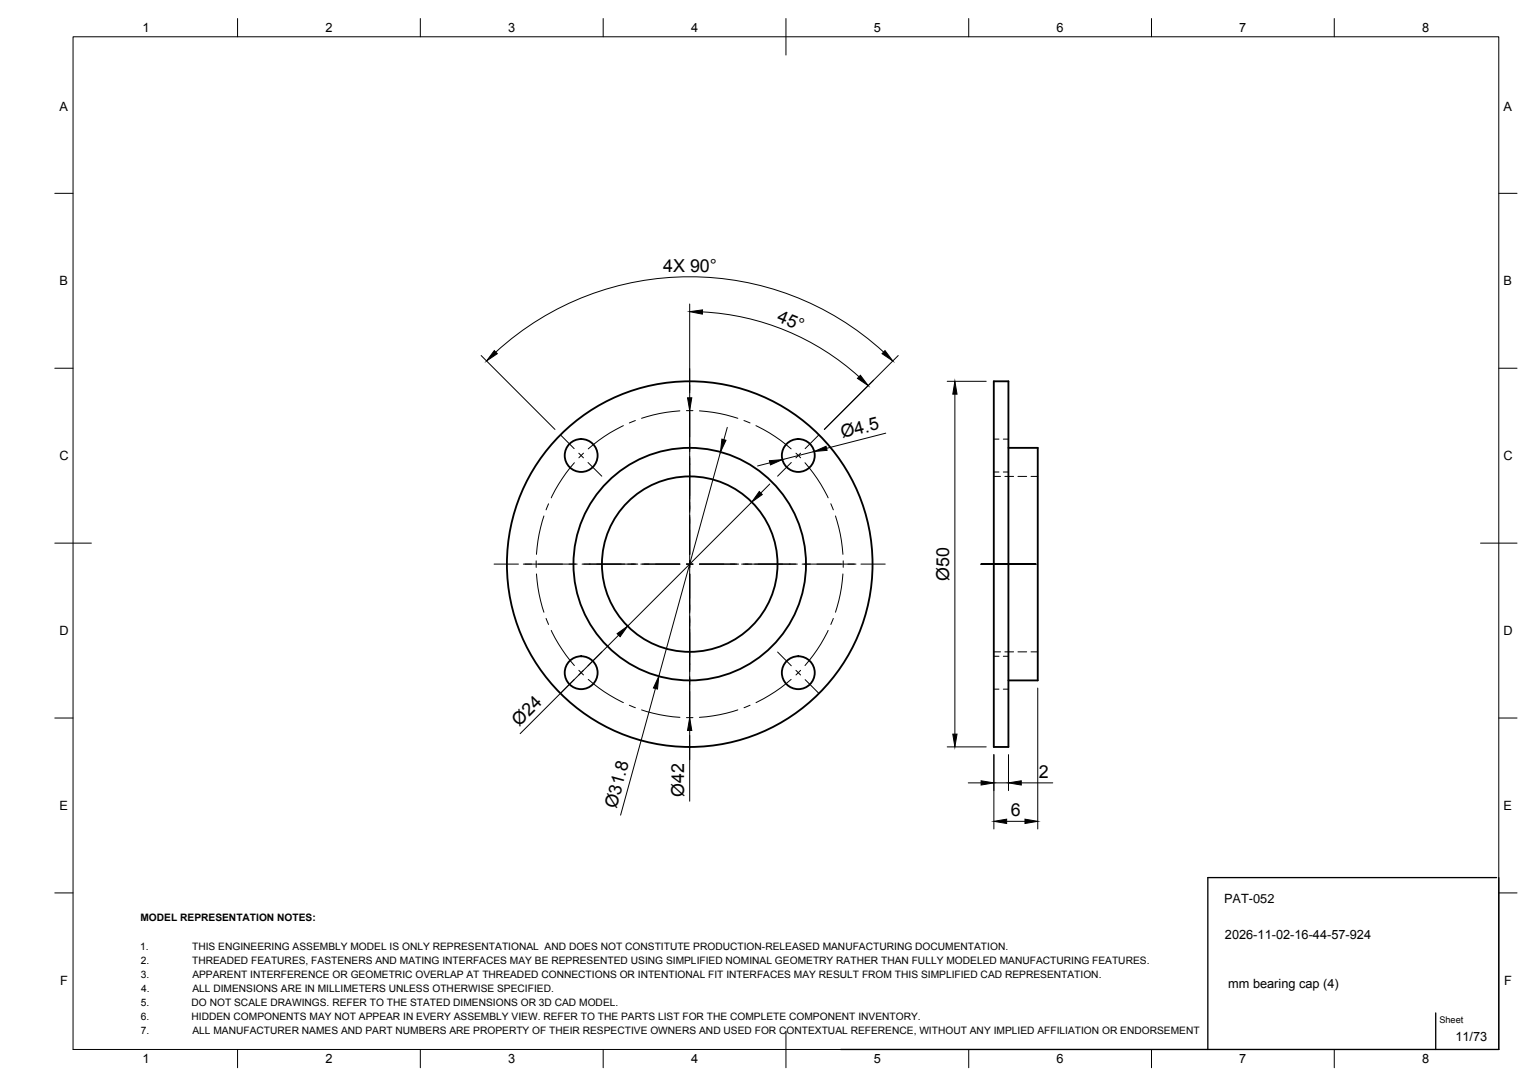
ISO-10303-21;
HEADER;
/* Generated by software containing ST-Developer
 * from STEP Tools, Inc. (www.steptools.com) 
 */

FILE_DESCRIPTION(
/* description */ ('Hand-crank gear train demonstrator'),
/* implementation_level */ '2;1');

FILE_NAME(
/* name */ 'mm bearing cap (4).step',
/* time_stamp */ '2026-10-28T03:22:13-07:00',
/* author */ (''),
/* organization */ (''),
/* preprocessor_version */ 'ST-DEVELOPER v20.2',
/* originating_system */ 'Autodesk Translation Framework v15.17.0.0',
/* authorisation */ '');

FILE_SCHEMA (('AUTOMOTIVE_DESIGN { 1 0 10303 214 3 1 1 }'));
ENDSEC;

DATA;
#10=MECHANICAL_DESIGN_GEOMETRIC_PRESENTATION_REPRESENTATION('',(#1196),#62758);
#1068=SHAPE_REPRESENTATION_RELATIONSHIP('SRR','None',#63040,#1132);
#1132=ADVANCED_BREP_SHAPE_REPRESENTATION('',(#1274),#62694);
#1196=STYLED_ITEM('',(#63462),#1274);
#1274=MANIFOLD_SOLID_BREP('Body1',#16377);
#1443=FACE_BOUND('',#3264,.T.);
#1444=FACE_BOUND('',#3268,.T.);
#1445=FACE_BOUND('',#3269,.T.);
#1446=FACE_BOUND('',#3270,.T.);
#1447=FACE_BOUND('',#3271,.T.);
#1448=FACE_BOUND('',#3272,.T.);
#1449=FACE_BOUND('',#3274,.T.);
#1450=FACE_BOUND('',#3275,.T.);
#1451=FACE_BOUND('',#3276,.T.);
#1452=FACE_BOUND('',#3277,.T.);
#1453=FACE_BOUND('',#3278,.T.);
#1670=PLANE('',#17400);
#1671=PLANE('',#17407);
#1672=PLANE('',#17408);
#2221=FACE_OUTER_BOUND('',#3258,.T.);
#2222=FACE_OUTER_BOUND('',#3259,.T.);
#2223=FACE_OUTER_BOUND('',#3260,.T.);
#2224=FACE_OUTER_BOUND('',#3261,.T.);
#2225=FACE_OUTER_BOUND('',#3262,.T.);
#2226=FACE_OUTER_BOUND('',#3263,.T.);
#2227=FACE_OUTER_BOUND('',#3265,.T.);
#2228=FACE_OUTER_BOUND('',#3266,.T.);
#2229=FACE_OUTER_BOUND('',#3267,.T.);
#2230=FACE_OUTER_BOUND('',#3273,.T.);
#3258=EDGE_LOOP('',(#11291,#11292,#11293,#11294));
#3259=EDGE_LOOP('',(#11295,#11296,#11297,#11298));
#3260=EDGE_LOOP('',(#11299,#11300,#11301,#11302));
#3261=EDGE_LOOP('',(#11303,#11304,#11305,#11306));
#3262=EDGE_LOOP('',(#11307,#11308,#11309,#11310));
#3263=EDGE_LOOP('',(#11311));
#3264=EDGE_LOOP('',(#11312));
#3265=EDGE_LOOP('',(#11313,#11314,#11315,#11316));
#3266=EDGE_LOOP('',(#11317,#11318,#11319,#11320));
#3267=EDGE_LOOP('',(#11321));
#3268=EDGE_LOOP('',(#11322));
#3269=EDGE_LOOP('',(#11323));
#3270=EDGE_LOOP('',(#11324));
#3271=EDGE_LOOP('',(#11325));
#3272=EDGE_LOOP('',(#11326));
#3273=EDGE_LOOP('',(#11327));
#3274=EDGE_LOOP('',(#11328));
#3275=EDGE_LOOP('',(#11329));
#3276=EDGE_LOOP('',(#11330));
#3277=EDGE_LOOP('',(#11331));
#3278=EDGE_LOOP('',(#11332));
#4395=LINE('',#23800,#5527);
#4396=LINE('',#23806,#5528);
#4397=LINE('',#23812,#5529);
#4398=LINE('',#23818,#5530);
#4399=LINE('',#23824,#5531);
#4400=LINE('',#23831,#5532);
#4401=LINE('',#23837,#5533);
#5527=VECTOR('',#19398,0.225);
#5528=VECTOR('',#19405,0.225);
#5529=VECTOR('',#19412,0.225);
#5530=VECTOR('',#19419,0.225);
#5531=VECTOR('',#19426,1.59);
#5532=VECTOR('',#19435,1.2);
#5533=VECTOR('',#19442,2.5);
#6669=CIRCLE('',#17386,0.225);
#6670=CIRCLE('',#17387,0.225);
#6671=CIRCLE('',#17389,0.225);
#6672=CIRCLE('',#17390,0.225);
#6673=CIRCLE('',#17392,0.225);
#6674=CIRCLE('',#17393,0.225);
#6675=CIRCLE('',#17395,0.225);
#6676=CIRCLE('',#17396,0.225);
#6677=CIRCLE('',#17398,1.59);
#6678=CIRCLE('',#17399,1.59);
#6679=CIRCLE('',#17401,1.2);
#6680=CIRCLE('',#17403,1.2);
#6681=CIRCLE('',#17405,2.5);
#6682=CIRCLE('',#17406,2.5);
#7363=VERTEX_POINT('',#23797);
#7364=VERTEX_POINT('',#23799);
#7365=VERTEX_POINT('',#23803);
#7366=VERTEX_POINT('',#23805);
#7367=VERTEX_POINT('',#23809);
#7368=VERTEX_POINT('',#23811);
#7369=VERTEX_POINT('',#23815);
#7370=VERTEX_POINT('',#23817);
#7371=VERTEX_POINT('',#23821);
#7372=VERTEX_POINT('',#23823);
#7373=VERTEX_POINT('',#23827);
#7374=VERTEX_POINT('',#23830);
#7375=VERTEX_POINT('',#23834);
#7376=VERTEX_POINT('',#23836);
#8897=EDGE_CURVE('',#7363,#7363,#6669,.T.);
#8898=EDGE_CURVE('',#7363,#7364,#4395,.T.);
#8899=EDGE_CURVE('',#7364,#7364,#6670,.T.);
#8900=EDGE_CURVE('',#7365,#7365,#6671,.T.);
#8901=EDGE_CURVE('',#7365,#7366,#4396,.T.);
#8902=EDGE_CURVE('',#7366,#7366,#6672,.T.);
#8903=EDGE_CURVE('',#7367,#7367,#6673,.T.);
#8904=EDGE_CURVE('',#7367,#7368,#4397,.T.);
#8905=EDGE_CURVE('',#7368,#7368,#6674,.T.);
#8906=EDGE_CURVE('',#7369,#7369,#6675,.T.);
#8907=EDGE_CURVE('',#7369,#7370,#4398,.T.);
#8908=EDGE_CURVE('',#7370,#7370,#6676,.T.);
#8909=EDGE_CURVE('',#7371,#7371,#6677,.T.);
#8910=EDGE_CURVE('',#7371,#7372,#4399,.T.);
#8911=EDGE_CURVE('',#7372,#7372,#6678,.T.);
#8912=EDGE_CURVE('',#7373,#7373,#6679,.T.);
#8913=EDGE_CURVE('',#7373,#7374,#4400,.T.);
#8914=EDGE_CURVE('',#7374,#7374,#6680,.T.);
#8915=EDGE_CURVE('',#7375,#7375,#6681,.T.);
#8916=EDGE_CURVE('',#7375,#7376,#4401,.T.);
#8917=EDGE_CURVE('',#7376,#7376,#6682,.T.);
#11291=ORIENTED_EDGE('',*,*,#8897,.F.);
#11292=ORIENTED_EDGE('',*,*,#8898,.T.);
#11293=ORIENTED_EDGE('',*,*,#8899,.F.);
#11294=ORIENTED_EDGE('',*,*,#8898,.F.);
#11295=ORIENTED_EDGE('',*,*,#8900,.F.);
#11296=ORIENTED_EDGE('',*,*,#8901,.T.);
#11297=ORIENTED_EDGE('',*,*,#8902,.F.);
#11298=ORIENTED_EDGE('',*,*,#8901,.F.);
#11299=ORIENTED_EDGE('',*,*,#8903,.F.);
#11300=ORIENTED_EDGE('',*,*,#8904,.T.);
#11301=ORIENTED_EDGE('',*,*,#8905,.F.);
#11302=ORIENTED_EDGE('',*,*,#8904,.F.);
#11303=ORIENTED_EDGE('',*,*,#8906,.F.);
#11304=ORIENTED_EDGE('',*,*,#8907,.T.);
#11305=ORIENTED_EDGE('',*,*,#8908,.F.);
#11306=ORIENTED_EDGE('',*,*,#8907,.F.);
#11307=ORIENTED_EDGE('',*,*,#8909,.F.);
#11308=ORIENTED_EDGE('',*,*,#8910,.T.);
#11309=ORIENTED_EDGE('',*,*,#8911,.F.);
#11310=ORIENTED_EDGE('',*,*,#8910,.F.);
#11311=ORIENTED_EDGE('',*,*,#8909,.T.);
#11312=ORIENTED_EDGE('',*,*,#8912,.T.);
#11313=ORIENTED_EDGE('',*,*,#8912,.F.);
#11314=ORIENTED_EDGE('',*,*,#8913,.T.);
#11315=ORIENTED_EDGE('',*,*,#8914,.T.);
#11316=ORIENTED_EDGE('',*,*,#8913,.F.);
#11317=ORIENTED_EDGE('',*,*,#8915,.F.);
#11318=ORIENTED_EDGE('',*,*,#8916,.T.);
#11319=ORIENTED_EDGE('',*,*,#8917,.T.);
#11320=ORIENTED_EDGE('',*,*,#8916,.F.);
#11321=ORIENTED_EDGE('',*,*,#8915,.T.);
#11322=ORIENTED_EDGE('',*,*,#8911,.T.);
#11323=ORIENTED_EDGE('',*,*,#8908,.T.);
#11324=ORIENTED_EDGE('',*,*,#8905,.T.);
#11325=ORIENTED_EDGE('',*,*,#8902,.T.);
#11326=ORIENTED_EDGE('',*,*,#8899,.T.);
#11327=ORIENTED_EDGE('',*,*,#8917,.F.);
#11328=ORIENTED_EDGE('',*,*,#8914,.F.);
#11329=ORIENTED_EDGE('',*,*,#8906,.T.);
#11330=ORIENTED_EDGE('',*,*,#8903,.T.);
#11331=ORIENTED_EDGE('',*,*,#8900,.T.);
#11332=ORIENTED_EDGE('',*,*,#8897,.T.);
#15225=CYLINDRICAL_SURFACE('',#17385,0.225);
#15226=CYLINDRICAL_SURFACE('',#17388,0.225);
#15227=CYLINDRICAL_SURFACE('',#17391,0.225);
#15228=CYLINDRICAL_SURFACE('',#17394,0.225);
#15229=CYLINDRICAL_SURFACE('',#17397,1.59);
#15230=CYLINDRICAL_SURFACE('',#17402,1.2);
#15231=CYLINDRICAL_SURFACE('',#17404,2.5);
#15531=ADVANCED_FACE('',(#2221),#15225,.F.);
#15532=ADVANCED_FACE('',(#2222),#15226,.F.);
#15533=ADVANCED_FACE('',(#2223),#15227,.F.);
#15534=ADVANCED_FACE('',(#2224),#15228,.F.);
#15535=ADVANCED_FACE('',(#2225),#15229,.T.);
#15536=ADVANCED_FACE('',(#2226,#1443),#1670,.T.);
#15537=ADVANCED_FACE('',(#2227),#15230,.F.);
#15538=ADVANCED_FACE('',(#2228),#15231,.T.);
#15539=ADVANCED_FACE('',(#2229,#1444,#1445,#1446,#1447,#1448),#1671,.T.);
#15540=ADVANCED_FACE('',(#2230,#1449,#1450,#1451,#1452,#1453),#1672,.F.);
#16377=CLOSED_SHELL('',(#15531,#15532,#15533,#15534,#15535,#15536,#15537,
#15538,#15539,#15540));
#17384=AXIS2_PLACEMENT_3D('',#23795,#19392,#19393);
#17385=AXIS2_PLACEMENT_3D('',#23796,#19394,#19395);
#17386=AXIS2_PLACEMENT_3D('',#23798,#19396,#19397);
#17387=AXIS2_PLACEMENT_3D('',#23801,#19399,#19400);
#17388=AXIS2_PLACEMENT_3D('',#23802,#19401,#19402);
#17389=AXIS2_PLACEMENT_3D('',#23804,#19403,#19404);
#17390=AXIS2_PLACEMENT_3D('',#23807,#19406,#19407);
#17391=AXIS2_PLACEMENT_3D('',#23808,#19408,#19409);
#17392=AXIS2_PLACEMENT_3D('',#23810,#19410,#19411);
#17393=AXIS2_PLACEMENT_3D('',#23813,#19413,#19414);
#17394=AXIS2_PLACEMENT_3D('',#23814,#19415,#19416);
#17395=AXIS2_PLACEMENT_3D('',#23816,#19417,#19418);
#17396=AXIS2_PLACEMENT_3D('',#23819,#19420,#19421);
#17397=AXIS2_PLACEMENT_3D('',#23820,#19422,#19423);
#17398=AXIS2_PLACEMENT_3D('',#23822,#19424,#19425);
#17399=AXIS2_PLACEMENT_3D('',#23825,#19427,#19428);
#17400=AXIS2_PLACEMENT_3D('',#23826,#19429,#19430);
#17401=AXIS2_PLACEMENT_3D('',#23828,#19431,#19432);
#17402=AXIS2_PLACEMENT_3D('',#23829,#19433,#19434);
#17403=AXIS2_PLACEMENT_3D('',#23832,#19436,#19437);
#17404=AXIS2_PLACEMENT_3D('',#23833,#19438,#19439);
#17405=AXIS2_PLACEMENT_3D('',#23835,#19440,#19441);
#17406=AXIS2_PLACEMENT_3D('',#23838,#19443,#19444);
#17407=AXIS2_PLACEMENT_3D('',#23839,#19445,#19446);
#17408=AXIS2_PLACEMENT_3D('',#23840,#19447,#19448);
#19392=DIRECTION('axis',(0.,0.,1.));
#19393=DIRECTION('refdir',(1.,0.,0.));
#19394=DIRECTION('center_axis',(0.,1.,0.));
#19395=DIRECTION('ref_axis',(1.,0.,0.));
#19396=DIRECTION('center_axis',(0.,1.,0.));
#19397=DIRECTION('ref_axis',(1.,0.,0.));
#19398=DIRECTION('',(0.,1.,0.));
#19399=DIRECTION('center_axis',(0.,-1.,0.));
#19400=DIRECTION('ref_axis',(1.,0.,0.));
#19401=DIRECTION('center_axis',(0.,1.,0.));
#19402=DIRECTION('ref_axis',(1.,0.,0.));
#19403=DIRECTION('center_axis',(0.,1.,0.));
#19404=DIRECTION('ref_axis',(1.,0.,0.));
#19405=DIRECTION('',(0.,1.,0.));
#19406=DIRECTION('center_axis',(0.,-1.,0.));
#19407=DIRECTION('ref_axis',(1.,0.,0.));
#19408=DIRECTION('center_axis',(0.,1.,0.));
#19409=DIRECTION('ref_axis',(1.,0.,0.));
#19410=DIRECTION('center_axis',(0.,1.,0.));
#19411=DIRECTION('ref_axis',(1.,0.,0.));
#19412=DIRECTION('',(0.,1.,0.));
#19413=DIRECTION('center_axis',(0.,-1.,0.));
#19414=DIRECTION('ref_axis',(1.,0.,0.));
#19415=DIRECTION('center_axis',(0.,1.,0.));
#19416=DIRECTION('ref_axis',(1.,0.,0.));
#19417=DIRECTION('center_axis',(0.,1.,0.));
#19418=DIRECTION('ref_axis',(1.,0.,0.));
#19419=DIRECTION('',(0.,1.,0.));
#19420=DIRECTION('center_axis',(0.,-1.,0.));
#19421=DIRECTION('ref_axis',(1.,0.,0.));
#19422=DIRECTION('center_axis',(0.,1.,0.));
#19423=DIRECTION('ref_axis',(1.,0.,0.));
#19424=DIRECTION('center_axis',(0.,1.,0.));
#19425=DIRECTION('ref_axis',(1.,0.,0.));
#19426=DIRECTION('',(0.,-1.,0.));
#19427=DIRECTION('center_axis',(0.,-1.,0.));
#19428=DIRECTION('ref_axis',(1.,0.,0.));
#19429=DIRECTION('center_axis',(0.,1.,0.));
#19430=DIRECTION('ref_axis',(1.,0.,0.));
#19431=DIRECTION('center_axis',(0.,-1.,0.));
#19432=DIRECTION('ref_axis',(1.,0.,0.));
#19433=DIRECTION('center_axis',(0.,1.,0.));
#19434=DIRECTION('ref_axis',(1.,0.,0.));
#19435=DIRECTION('',(0.,-1.,0.));
#19436=DIRECTION('center_axis',(0.,-1.,0.));
#19437=DIRECTION('ref_axis',(1.,0.,0.));
#19438=DIRECTION('center_axis',(0.,1.,0.));
#19439=DIRECTION('ref_axis',(1.,0.,0.));
#19440=DIRECTION('center_axis',(0.,1.,0.));
#19441=DIRECTION('ref_axis',(1.,0.,0.));
#19442=DIRECTION('',(0.,-1.,0.));
#19443=DIRECTION('center_axis',(0.,1.,0.));
#19444=DIRECTION('ref_axis',(1.,0.,0.));
#19445=DIRECTION('center_axis',(0.,1.,0.));
#19446=DIRECTION('ref_axis',(1.,0.,0.));
#19447=DIRECTION('center_axis',(0.,1.,0.));
#19448=DIRECTION('ref_axis',(1.,0.,0.));
#23795=CARTESIAN_POINT('',(0.,0.,0.));
#23796=CARTESIAN_POINT('Origin',(10.5150757595082,-2.7,7.51507575950825));
#23797=CARTESIAN_POINT('',(10.2900757595082,-2.6,7.51507575950825));
#23798=CARTESIAN_POINT('Origin',(10.5150757595082,-2.6,7.51507575950825));
#23799=CARTESIAN_POINT('',(10.2900757595082,-2.4,7.51507575950825));
#23800=CARTESIAN_POINT('',(10.2900757595082,-2.7,7.51507575950825));
#23801=CARTESIAN_POINT('Origin',(10.5150757595082,-2.4,7.51507575950825));
#23802=CARTESIAN_POINT('Origin',(10.5150757595082,-2.7,10.4849242404918));
#23803=CARTESIAN_POINT('',(10.2900757595082,-2.6,10.4849242404918));
#23804=CARTESIAN_POINT('Origin',(10.5150757595082,-2.6,10.4849242404918));
#23805=CARTESIAN_POINT('',(10.2900757595082,-2.4,10.4849242404918));
#23806=CARTESIAN_POINT('',(10.2900757595082,-2.7,10.4849242404918));
#23807=CARTESIAN_POINT('Origin',(10.5150757595082,-2.4,10.4849242404918));
#23808=CARTESIAN_POINT('Origin',(13.4849242404918,-2.7,10.4849242404918));
#23809=CARTESIAN_POINT('',(13.2599242404918,-2.6,10.4849242404918));
#23810=CARTESIAN_POINT('Origin',(13.4849242404918,-2.6,10.4849242404918));
#23811=CARTESIAN_POINT('',(13.2599242404918,-2.4,10.4849242404918));
#23812=CARTESIAN_POINT('',(13.2599242404918,-2.7,10.4849242404918));
#23813=CARTESIAN_POINT('Origin',(13.4849242404918,-2.4,10.4849242404918));
#23814=CARTESIAN_POINT('Origin',(13.4849242404918,-2.7,7.51507575950825));
#23815=CARTESIAN_POINT('',(13.2599242404918,-2.6,7.51507575950825));
#23816=CARTESIAN_POINT('Origin',(13.4849242404918,-2.6,7.51507575950825));
#23817=CARTESIAN_POINT('',(13.2599242404918,-2.4,7.51507575950825));
#23818=CARTESIAN_POINT('',(13.2599242404918,-2.7,7.51507575950825));
#23819=CARTESIAN_POINT('Origin',(13.4849242404918,-2.4,7.51507575950825));
#23820=CARTESIAN_POINT('Origin',(12.,-2.4,9.));
#23821=CARTESIAN_POINT('',(10.41,-2.,9.));
#23822=CARTESIAN_POINT('Origin',(12.,-2.,9.));
#23823=CARTESIAN_POINT('',(10.41,-2.4,9.));
#23824=CARTESIAN_POINT('',(10.41,-2.4,9.));
#23825=CARTESIAN_POINT('Origin',(12.,-2.4,9.));
#23826=CARTESIAN_POINT('Origin',(12.,-2.,9.));
#23827=CARTESIAN_POINT('',(10.8,-2.,9.));
#23828=CARTESIAN_POINT('Origin',(12.,-2.,9.));
#23829=CARTESIAN_POINT('Origin',(12.,-2.6,9.));
#23830=CARTESIAN_POINT('',(10.8,-2.6,9.));
#23831=CARTESIAN_POINT('',(10.8,-2.6,9.));
#23832=CARTESIAN_POINT('Origin',(12.,-2.6,9.));
#23833=CARTESIAN_POINT('Origin',(12.,-2.6,9.));
#23834=CARTESIAN_POINT('',(9.5,-2.4,9.));
#23835=CARTESIAN_POINT('Origin',(12.,-2.4,9.));
#23836=CARTESIAN_POINT('',(9.5,-2.6,9.));
#23837=CARTESIAN_POINT('',(9.5,-2.6,9.));
#23838=CARTESIAN_POINT('Origin',(12.,-2.6,9.));
#23839=CARTESIAN_POINT('Origin',(12.,-2.4,9.));
#23840=CARTESIAN_POINT('Origin',(12.,-2.6,9.));
#62620=UNCERTAINTY_MEASURE_WITH_UNIT(LENGTH_MEASURE(0.001),#62759,
'DISTANCE_ACCURACY_VALUE',
'Maximum model space distance between geometric entities at asserted c
onnectivities');
#62684=UNCERTAINTY_MEASURE_WITH_UNIT(LENGTH_MEASURE(0.001),#62759,
'DISTANCE_ACCURACY_VALUE',
'Maximum model space distance between geometric entities at asserted c
onnectivities');
#62694=(
GEOMETRIC_REPRESENTATION_CONTEXT(3)
GLOBAL_UNCERTAINTY_ASSIGNED_CONTEXT((#62620))
GLOBAL_UNIT_ASSIGNED_CONTEXT((#62759,#62761,#62762))
REPRESENTATION_CONTEXT('','3D')
);
#62758=(
GEOMETRIC_REPRESENTATION_CONTEXT(3)
GLOBAL_UNCERTAINTY_ASSIGNED_CONTEXT((#62684))
GLOBAL_UNIT_ASSIGNED_CONTEXT((#62759,#62761,#62762))
REPRESENTATION_CONTEXT('','3D')
);
#62759=(
LENGTH_UNIT()
NAMED_UNIT(*)
SI_UNIT(.CENTI.,.METRE.)
);
#62761=(
NAMED_UNIT(*)
PLANE_ANGLE_UNIT()
SI_UNIT($,.RADIAN.)
);
#62762=(
NAMED_UNIT(*)
SI_UNIT($,.STERADIAN.)
SOLID_ANGLE_UNIT()
);
#62772=SHAPE_DEFINITION_REPRESENTATION(#62845,#63040);
#62845=PRODUCT_DEFINITION_SHAPE('',$,#63114);
#63040=SHAPE_REPRESENTATION('',(#17384),#62694);
#63104=PRODUCT_DEFINITION_CONTEXT('part definition',#63325,'design');
#63114=PRODUCT_DEFINITION('mm bearing cap (4)','mm bearing cap (4)',#63187,
#63104);
#63187=PRODUCT_DEFINITION_FORMATION('',$,#63336);
#63325=APPLICATION_CONTEXT(
'Core Data for Automotive Mechanical Design Process');
#63326=PRODUCT_CONTEXT('part definition',#63325,'mechanical');
#63336=PRODUCT('mm bearing cap (4)','mm bearing cap (4)','mm bearing cap (4)',
(#63326));
#63456=COLOUR_RGB('Grey',0.48,0.52,0.57);
#63457=FILL_AREA_STYLE_COLOUR('',#63456);
#63458=FILL_AREA_STYLE('',(#63457));
#63459=SURFACE_STYLE_FILL_AREA(#63458);
#63460=SURFACE_SIDE_STYLE('',(#63459));
#63461=SURFACE_STYLE_USAGE(.BOTH.,#63460);
#63462=PRESENTATION_STYLE_ASSIGNMENT((#63461));
ENDSEC;
END-ISO-10303-21;
